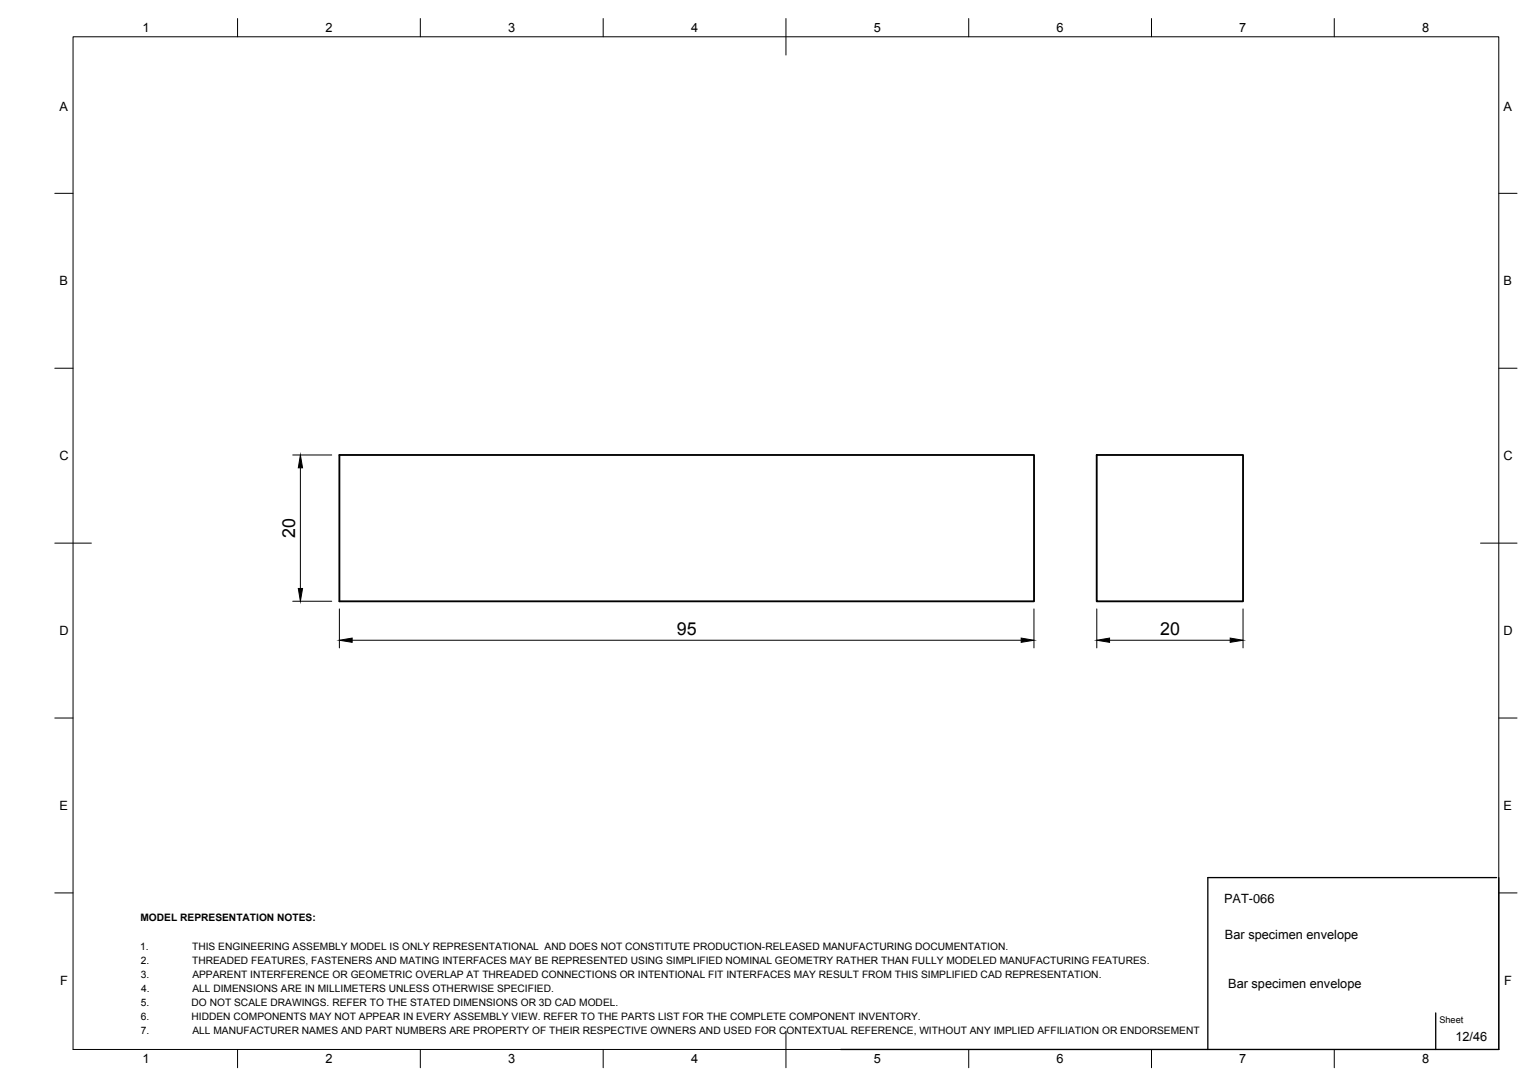
ISO-10303-21;
HEADER;
/* Generated by software containing ST-Developer
 * from STEP Tools, Inc. (www.steptools.com) 
 */

FILE_DESCRIPTION(
/* description */ ('Lever-operated bar clamp (toggle)'),
/* implementation_level */ '2;1');

FILE_NAME(
/* name */ 'Bar specimen envelope.step',
/* time_stamp */ '2026-10-28T03:25:02-07:00',
/* author */ (''),
/* organization */ (''),
/* preprocessor_version */ 'ST-DEVELOPER v20.2',
/* originating_system */ 'Autodesk Translation Framework v15.17.0.0',
/* authorisation */ '');

FILE_SCHEMA (('AUTOMOTIVE_DESIGN { 1 0 10303 214 3 1 1 }'));
ENDSEC;

DATA;
#10=MECHANICAL_DESIGN_GEOMETRIC_PRESENTATION_REPRESENTATION('',(#417),#12413);
#341=SHAPE_REPRESENTATION_RELATIONSHIP('SRR','None',#12580,#379);
#379=ADVANCED_BREP_SHAPE_REPRESENTATION('',(#464),#12377);
#417=STYLED_ITEM('',(#12883),#464);
#464=MANIFOLD_SOLID_BREP('Body1',#6576);
#702=PLANE('',#7253);
#703=PLANE('',#7254);
#704=PLANE('',#7255);
#705=PLANE('',#7256);
#706=PLANE('',#7257);
#707=PLANE('',#7258);
#990=FACE_OUTER_BOUND('',#1477,.T.);
#991=FACE_OUTER_BOUND('',#1478,.T.);
#992=FACE_OUTER_BOUND('',#1479,.T.);
#993=FACE_OUTER_BOUND('',#1480,.T.);
#994=FACE_OUTER_BOUND('',#1481,.T.);
#995=FACE_OUTER_BOUND('',#1482,.T.);
#1477=EDGE_LOOP('',(#4871,#4872,#4873,#4874));
#1478=EDGE_LOOP('',(#4875,#4876,#4877,#4878));
#1479=EDGE_LOOP('',(#4879,#4880,#4881,#4882));
#1480=EDGE_LOOP('',(#4883,#4884,#4885,#4886));
#1481=EDGE_LOOP('',(#4887,#4888,#4889,#4890));
#1482=EDGE_LOOP('',(#4891,#4892,#4893,#4894));
#1974=LINE('',#10535,#2415);
#1975=LINE('',#10537,#2416);
#1976=LINE('',#10539,#2417);
#1977=LINE('',#10540,#2418);
#1978=LINE('',#10543,#2419);
#1979=LINE('',#10545,#2420);
#1980=LINE('',#10546,#2421);
#1981=LINE('',#10549,#2422);
#1982=LINE('',#10551,#2423);
#1983=LINE('',#10552,#2424);
#1984=LINE('',#10554,#2425);
#1985=LINE('',#10555,#2426);
#2415=VECTOR('',#8447,1.);
#2416=VECTOR('',#8448,1.);
#2417=VECTOR('',#8449,1.);
#2418=VECTOR('',#8450,1.);
#2419=VECTOR('',#8453,1.);
#2420=VECTOR('',#8454,1.);
#2421=VECTOR('',#8455,1.);
#2422=VECTOR('',#8458,1.);
#2423=VECTOR('',#8459,1.);
#2424=VECTOR('',#8460,1.);
#2425=VECTOR('',#8463,1.);
#2426=VECTOR('',#8464,1.);
#3224=VERTEX_POINT('',#10533);
#3225=VERTEX_POINT('',#10534);
#3226=VERTEX_POINT('',#10536);
#3227=VERTEX_POINT('',#10538);
#3228=VERTEX_POINT('',#10542);
#3229=VERTEX_POINT('',#10544);
#3230=VERTEX_POINT('',#10548);
#3231=VERTEX_POINT('',#10550);
#3840=EDGE_CURVE('',#3224,#3225,#1974,.T.);
#3841=EDGE_CURVE('',#3225,#3226,#1975,.T.);
#3842=EDGE_CURVE('',#3227,#3226,#1976,.T.);
#3843=EDGE_CURVE('',#3224,#3227,#1977,.T.);
#3844=EDGE_CURVE('',#3228,#3224,#1978,.T.);
#3845=EDGE_CURVE('',#3229,#3227,#1979,.T.);
#3846=EDGE_CURVE('',#3228,#3229,#1980,.T.);
#3847=EDGE_CURVE('',#3230,#3228,#1981,.T.);
#3848=EDGE_CURVE('',#3231,#3229,#1982,.T.);
#3849=EDGE_CURVE('',#3230,#3231,#1983,.T.);
#3850=EDGE_CURVE('',#3225,#3230,#1984,.T.);
#3851=EDGE_CURVE('',#3226,#3231,#1985,.T.);
#4871=ORIENTED_EDGE('',*,*,#3840,.T.);
#4872=ORIENTED_EDGE('',*,*,#3841,.T.);
#4873=ORIENTED_EDGE('',*,*,#3842,.F.);
#4874=ORIENTED_EDGE('',*,*,#3843,.F.);
#4875=ORIENTED_EDGE('',*,*,#3844,.T.);
#4876=ORIENTED_EDGE('',*,*,#3843,.T.);
#4877=ORIENTED_EDGE('',*,*,#3845,.F.);
#4878=ORIENTED_EDGE('',*,*,#3846,.F.);
#4879=ORIENTED_EDGE('',*,*,#3847,.T.);
#4880=ORIENTED_EDGE('',*,*,#3846,.T.);
#4881=ORIENTED_EDGE('',*,*,#3848,.F.);
#4882=ORIENTED_EDGE('',*,*,#3849,.F.);
#4883=ORIENTED_EDGE('',*,*,#3850,.T.);
#4884=ORIENTED_EDGE('',*,*,#3849,.T.);
#4885=ORIENTED_EDGE('',*,*,#3851,.F.);
#4886=ORIENTED_EDGE('',*,*,#3841,.F.);
#4887=ORIENTED_EDGE('',*,*,#3851,.T.);
#4888=ORIENTED_EDGE('',*,*,#3848,.T.);
#4889=ORIENTED_EDGE('',*,*,#3845,.T.);
#4890=ORIENTED_EDGE('',*,*,#3842,.T.);
#4891=ORIENTED_EDGE('',*,*,#3850,.F.);
#4892=ORIENTED_EDGE('',*,*,#3840,.F.);
#4893=ORIENTED_EDGE('',*,*,#3844,.F.);
#4894=ORIENTED_EDGE('',*,*,#3847,.F.);
#6265=ADVANCED_FACE('',(#990),#702,.T.);
#6266=ADVANCED_FACE('',(#991),#703,.T.);
#6267=ADVANCED_FACE('',(#992),#704,.T.);
#6268=ADVANCED_FACE('',(#993),#705,.T.);
#6269=ADVANCED_FACE('',(#994),#706,.T.);
#6270=ADVANCED_FACE('',(#995),#707,.F.);
#6576=CLOSED_SHELL('',(#6265,#6266,#6267,#6268,#6269,#6270));
#7252=AXIS2_PLACEMENT_3D('',#10531,#8443,#8444);
#7253=AXIS2_PLACEMENT_3D('',#10532,#8445,#8446);
#7254=AXIS2_PLACEMENT_3D('',#10541,#8451,#8452);
#7255=AXIS2_PLACEMENT_3D('',#10547,#8456,#8457);
#7256=AXIS2_PLACEMENT_3D('',#10553,#8461,#8462);
#7257=AXIS2_PLACEMENT_3D('',#10556,#8465,#8466);
#7258=AXIS2_PLACEMENT_3D('',#10557,#8467,#8468);
#8443=DIRECTION('axis',(0.,0.,1.));
#8444=DIRECTION('refdir',(1.,0.,0.));
#8445=DIRECTION('center_axis',(0.,1.,0.));
#8446=DIRECTION('ref_axis',(-1.,0.,0.));
#8447=DIRECTION('',(-1.,0.,0.));
#8448=DIRECTION('',(0.,0.,1.));
#8449=DIRECTION('',(-1.,0.,0.));
#8450=DIRECTION('',(0.,0.,1.));
#8451=DIRECTION('center_axis',(1.,0.,0.));
#8452=DIRECTION('ref_axis',(0.,1.,0.));
#8453=DIRECTION('',(0.,1.,0.));
#8454=DIRECTION('',(0.,1.,0.));
#8455=DIRECTION('',(0.,0.,1.));
#8456=DIRECTION('center_axis',(0.,-1.,0.));
#8457=DIRECTION('ref_axis',(1.,0.,0.));
#8458=DIRECTION('',(1.,0.,0.));
#8459=DIRECTION('',(1.,0.,0.));
#8460=DIRECTION('',(0.,0.,1.));
#8461=DIRECTION('center_axis',(-1.,0.,0.));
#8462=DIRECTION('ref_axis',(0.,-1.,0.));
#8463=DIRECTION('',(0.,-1.,0.));
#8464=DIRECTION('',(0.,-1.,0.));
#8465=DIRECTION('center_axis',(0.,0.,1.));
#8466=DIRECTION('ref_axis',(1.,0.,0.));
#8467=DIRECTION('center_axis',(0.,0.,1.));
#8468=DIRECTION('ref_axis',(1.,0.,0.));
#10531=CARTESIAN_POINT('',(0.,0.,0.));
#10532=CARTESIAN_POINT('Origin',(1.,3.5,1.));
#10533=CARTESIAN_POINT('',(1.,3.5,1.));
#10534=CARTESIAN_POINT('',(-1.,3.5,1.));
#10535=CARTESIAN_POINT('',(1.,3.5,1.));
#10536=CARTESIAN_POINT('',(-1.,3.5,3.));
#10537=CARTESIAN_POINT('',(-1.,3.5,1.));
#10538=CARTESIAN_POINT('',(1.,3.5,3.));
#10539=CARTESIAN_POINT('',(1.,3.5,3.));
#10540=CARTESIAN_POINT('',(1.,3.5,1.));
#10541=CARTESIAN_POINT('Origin',(1.,-6.,1.));
#10542=CARTESIAN_POINT('',(1.,-6.,1.));
#10543=CARTESIAN_POINT('',(1.,-6.,1.));
#10544=CARTESIAN_POINT('',(1.,-6.,3.));
#10545=CARTESIAN_POINT('',(1.,-6.,3.));
#10546=CARTESIAN_POINT('',(1.,-6.,1.));
#10547=CARTESIAN_POINT('Origin',(-1.,-6.,1.));
#10548=CARTESIAN_POINT('',(-1.,-6.,1.));
#10549=CARTESIAN_POINT('',(-1.,-6.,1.));
#10550=CARTESIAN_POINT('',(-1.,-6.,3.));
#10551=CARTESIAN_POINT('',(-1.,-6.,3.));
#10552=CARTESIAN_POINT('',(-1.,-6.,1.));
#10553=CARTESIAN_POINT('Origin',(-1.,3.5,1.));
#10554=CARTESIAN_POINT('',(-1.,3.5,1.));
#10555=CARTESIAN_POINT('',(-1.,3.5,3.));
#10556=CARTESIAN_POINT('Origin',(0.,-1.25,3.));
#10557=CARTESIAN_POINT('Origin',(0.,-1.25,1.));
#12331=UNCERTAINTY_MEASURE_WITH_UNIT(LENGTH_MEASURE(0.001),#12414,
'DISTANCE_ACCURACY_VALUE',
'Maximum model space distance between geometric entities at asserted c
onnectivities');
#12367=UNCERTAINTY_MEASURE_WITH_UNIT(LENGTH_MEASURE(0.001),#12414,
'DISTANCE_ACCURACY_VALUE',
'Maximum model space distance between geometric entities at asserted c
onnectivities');
#12377=(
GEOMETRIC_REPRESENTATION_CONTEXT(3)
GLOBAL_UNCERTAINTY_ASSIGNED_CONTEXT((#12331))
GLOBAL_UNIT_ASSIGNED_CONTEXT((#12414,#12416,#12417))
REPRESENTATION_CONTEXT('','3D')
);
#12413=(
GEOMETRIC_REPRESENTATION_CONTEXT(3)
GLOBAL_UNCERTAINTY_ASSIGNED_CONTEXT((#12367))
GLOBAL_UNIT_ASSIGNED_CONTEXT((#12414,#12416,#12417))
REPRESENTATION_CONTEXT('','3D')
);
#12414=(
LENGTH_UNIT()
NAMED_UNIT(*)
SI_UNIT(.CENTI.,.METRE.)
);
#12416=(
NAMED_UNIT(*)
PLANE_ANGLE_UNIT()
SI_UNIT($,.RADIAN.)
);
#12417=(
NAMED_UNIT(*)
SI_UNIT($,.STERADIAN.)
SOLID_ANGLE_UNIT()
);
#12427=SHAPE_DEFINITION_REPRESENTATION(#12472,#12580);
#12472=PRODUCT_DEFINITION_SHAPE('',$,#12626);
#12580=SHAPE_REPRESENTATION('',(#7252),#12377);
#12616=PRODUCT_DEFINITION_CONTEXT('part definition',#12753,'design');
#12626=PRODUCT_DEFINITION('Bar specimen envelope',
'Bar specimen envelope',#12671,#12616);
#12671=PRODUCT_DEFINITION_FORMATION('',$,#12764);
#12753=APPLICATION_CONTEXT(
'Core Data for Automotive Mechanical Design Process');
#12754=PRODUCT_CONTEXT('part definition',#12753,'mechanical');
#12764=PRODUCT('Bar specimen envelope','Bar specimen envelope',
'Bar specimen envelope',(#12754));
#12877=COLOUR_RGB('Off White',0.89,0.88,0.83);
#12878=FILL_AREA_STYLE_COLOUR('',#12877);
#12879=FILL_AREA_STYLE('',(#12878));
#12880=SURFACE_STYLE_FILL_AREA(#12879);
#12881=SURFACE_SIDE_STYLE('',(#12880));
#12882=SURFACE_STYLE_USAGE(.BOTH.,#12881);
#12883=PRESENTATION_STYLE_ASSIGNMENT((#12882));
ENDSEC;
END-ISO-10303-21;
